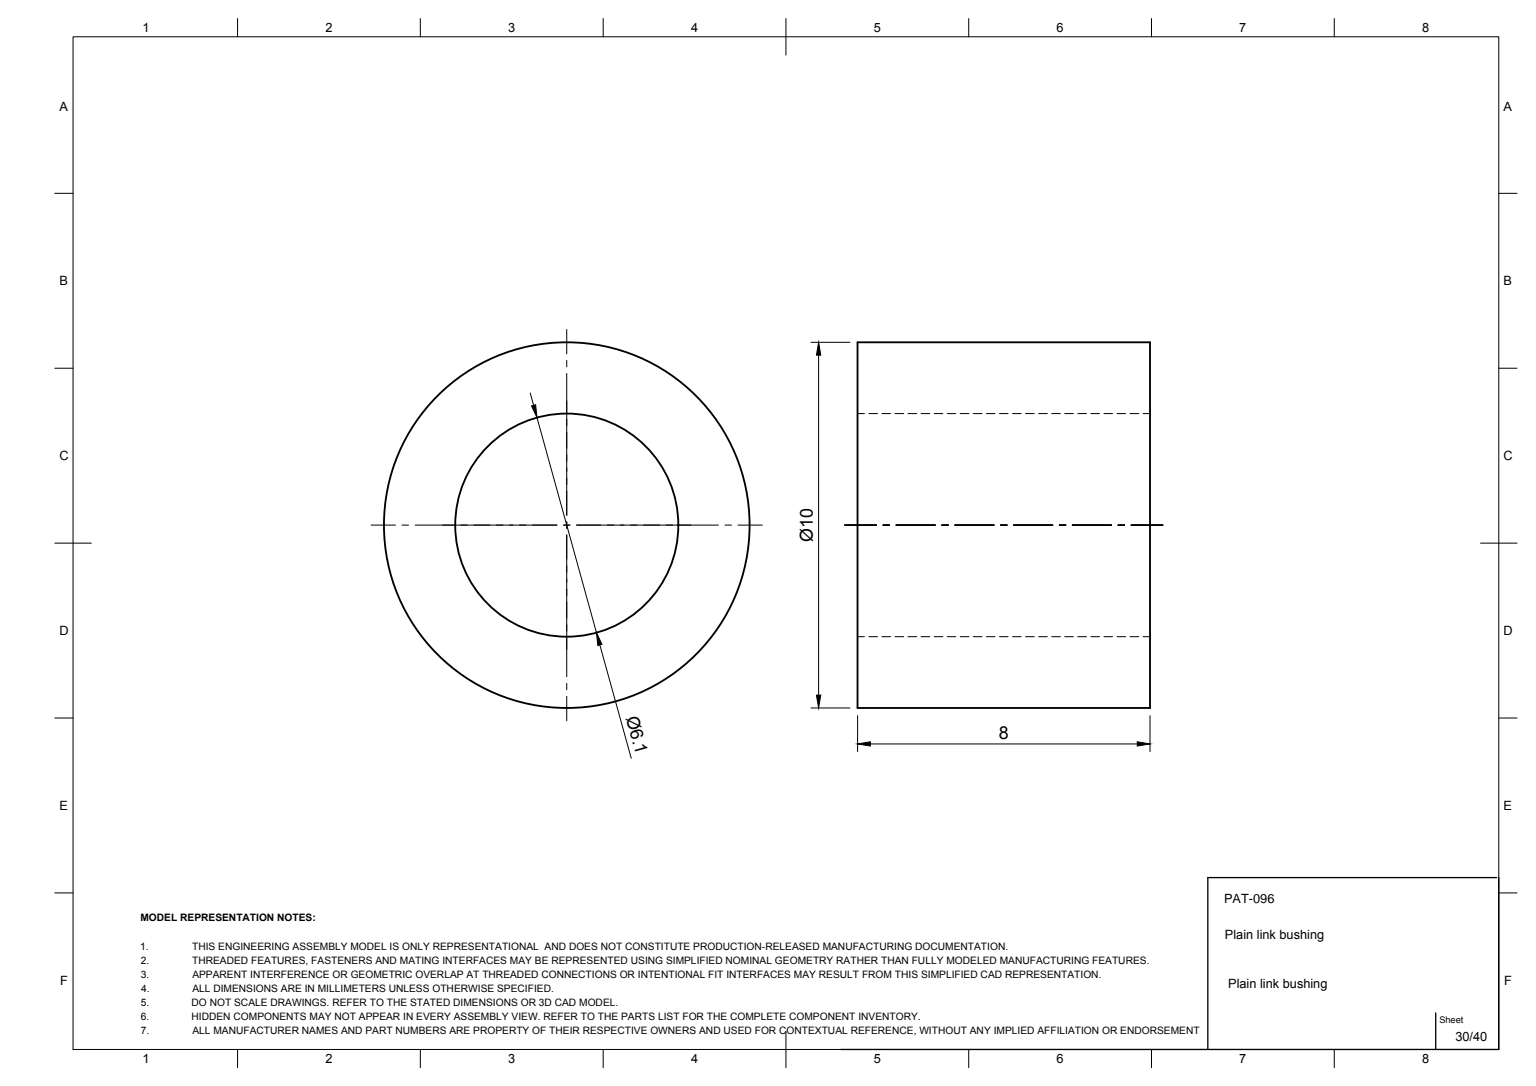
ISO-10303-21;
HEADER;
/* Generated by software containing ST-Developer
 * from STEP Tools, Inc. (www.steptools.com) 
 */

FILE_DESCRIPTION(
/* description */ ('PAT-096'),
/* implementation_level */ '2;1');

FILE_NAME(
/* name */ 'Plain link bushing.step',
/* time_stamp */ '2026-10-29T17:03:14-07:00',
/* author */ (''),
/* organization */ (''),
/* preprocessor_version */ 'ST-DEVELOPER v20.2',
/* originating_system */ 'Autodesk Translation Framework v15.17.0.0',
/* authorisation */ '');

FILE_SCHEMA (('AUTOMOTIVE_DESIGN { 1 0 10303 214 3 1 1 }'));
ENDSEC;

DATA;
#10=MECHANICAL_DESIGN_GEOMETRIC_PRESENTATION_REPRESENTATION('',(#427),#10650);
#357=SHAPE_REPRESENTATION_RELATIONSHIP('SRR','None',#10820,#388);
#388=ADVANCED_BREP_SHAPE_REPRESENTATION('',(#464),#10638);
#427=STYLED_ITEM('',(#11057),#464);
#464=MANIFOLD_SOLID_BREP('Body1',#5562);
#568=FACE_BOUND('',#1470,.T.);
#569=FACE_BOUND('',#1472,.T.);
#736=PLANE('',#6443);
#737=PLANE('',#6444);
#1036=FACE_OUTER_BOUND('',#1467,.T.);
#1037=FACE_OUTER_BOUND('',#1468,.T.);
#1038=FACE_OUTER_BOUND('',#1469,.T.);
#1039=FACE_OUTER_BOUND('',#1471,.T.);
#1467=EDGE_LOOP('',(#4731,#4732,#4733,#4734));
#1468=EDGE_LOOP('',(#4735,#4736,#4737,#4738));
#1469=EDGE_LOOP('',(#4739));
#1470=EDGE_LOOP('',(#4740));
#1471=EDGE_LOOP('',(#4741));
#1472=EDGE_LOOP('',(#4742));
#1834=LINE('',#10134,#2163);
#1835=LINE('',#10140,#2164);
#2163=VECTOR('',#7952,0.305);
#2164=VECTOR('',#7959,0.5);
#2503=CIRCLE('',#6438,0.305);
#2504=CIRCLE('',#6439,0.305);
#2505=CIRCLE('',#6441,0.5);
#2506=CIRCLE('',#6442,0.5);
#2923=VERTEX_POINT('',#10131);
#2924=VERTEX_POINT('',#10133);
#2925=VERTEX_POINT('',#10137);
#2926=VERTEX_POINT('',#10139);
#3544=EDGE_CURVE('',#2923,#2923,#2503,.T.);
#3545=EDGE_CURVE('',#2923,#2924,#1834,.T.);
#3546=EDGE_CURVE('',#2924,#2924,#2504,.T.);
#3547=EDGE_CURVE('',#2925,#2925,#2505,.T.);
#3548=EDGE_CURVE('',#2925,#2926,#1835,.T.);
#3549=EDGE_CURVE('',#2926,#2926,#2506,.T.);
#4731=ORIENTED_EDGE('',*,*,#3544,.F.);
#4732=ORIENTED_EDGE('',*,*,#3545,.T.);
#4733=ORIENTED_EDGE('',*,*,#3546,.T.);
#4734=ORIENTED_EDGE('',*,*,#3545,.F.);
#4735=ORIENTED_EDGE('',*,*,#3547,.F.);
#4736=ORIENTED_EDGE('',*,*,#3548,.T.);
#4737=ORIENTED_EDGE('',*,*,#3549,.T.);
#4738=ORIENTED_EDGE('',*,*,#3548,.F.);
#4739=ORIENTED_EDGE('',*,*,#3547,.T.);
#4740=ORIENTED_EDGE('',*,*,#3544,.T.);
#4741=ORIENTED_EDGE('',*,*,#3549,.F.);
#4742=ORIENTED_EDGE('',*,*,#3546,.F.);
#5162=CYLINDRICAL_SURFACE('',#6437,0.305);
#5163=CYLINDRICAL_SURFACE('',#6440,0.5);
#5441=ADVANCED_FACE('',(#1036),#5162,.F.);
#5442=ADVANCED_FACE('',(#1037),#5163,.T.);
#5443=ADVANCED_FACE('',(#1038,#568),#736,.T.);
#5444=ADVANCED_FACE('',(#1039,#569),#737,.F.);
#5562=CLOSED_SHELL('',(#5441,#5442,#5443,#5444));
#6436=AXIS2_PLACEMENT_3D('',#10129,#7946,#7947);
#6437=AXIS2_PLACEMENT_3D('',#10130,#7948,#7949);
#6438=AXIS2_PLACEMENT_3D('',#10132,#7950,#7951);
#6439=AXIS2_PLACEMENT_3D('',#10135,#7953,#7954);
#6440=AXIS2_PLACEMENT_3D('',#10136,#7955,#7956);
#6441=AXIS2_PLACEMENT_3D('',#10138,#7957,#7958);
#6442=AXIS2_PLACEMENT_3D('',#10141,#7960,#7961);
#6443=AXIS2_PLACEMENT_3D('',#10142,#7962,#7963);
#6444=AXIS2_PLACEMENT_3D('',#10143,#7964,#7965);
#7946=DIRECTION('axis',(0.,0.,1.));
#7947=DIRECTION('refdir',(1.,0.,0.));
#7948=DIRECTION('center_axis',(0.,0.,1.));
#7949=DIRECTION('ref_axis',(1.,0.,0.));
#7950=DIRECTION('center_axis',(0.,0.,-1.));
#7951=DIRECTION('ref_axis',(1.,0.,0.));
#7952=DIRECTION('',(0.,0.,-1.));
#7953=DIRECTION('center_axis',(0.,0.,-1.));
#7954=DIRECTION('ref_axis',(1.,0.,0.));
#7955=DIRECTION('center_axis',(0.,0.,1.));
#7956=DIRECTION('ref_axis',(1.,0.,0.));
#7957=DIRECTION('center_axis',(0.,0.,1.));
#7958=DIRECTION('ref_axis',(1.,0.,0.));
#7959=DIRECTION('',(0.,0.,-1.));
#7960=DIRECTION('center_axis',(0.,0.,1.));
#7961=DIRECTION('ref_axis',(1.,0.,0.));
#7962=DIRECTION('center_axis',(0.,0.,1.));
#7963=DIRECTION('ref_axis',(1.,0.,0.));
#7964=DIRECTION('center_axis',(0.,0.,1.));
#7965=DIRECTION('ref_axis',(1.,0.,0.));
#10129=CARTESIAN_POINT('',(0.,0.,0.));
#10130=CARTESIAN_POINT('Origin',(0.,2.,8.8));
#10131=CARTESIAN_POINT('',(-0.305,2.,9.6));
#10132=CARTESIAN_POINT('Origin',(0.,2.,9.6));
#10133=CARTESIAN_POINT('',(-0.305,2.,8.8));
#10134=CARTESIAN_POINT('',(-0.305,2.,8.8));
#10135=CARTESIAN_POINT('Origin',(0.,2.,8.8));
#10136=CARTESIAN_POINT('Origin',(0.,2.,8.8));
#10137=CARTESIAN_POINT('',(-0.5,2.,9.6));
#10138=CARTESIAN_POINT('Origin',(0.,2.,9.6));
#10139=CARTESIAN_POINT('',(-0.5,2.,8.8));
#10140=CARTESIAN_POINT('',(-0.5,2.,8.8));
#10141=CARTESIAN_POINT('Origin',(0.,2.,8.8));
#10142=CARTESIAN_POINT('Origin',(0.,2.,9.6));
#10143=CARTESIAN_POINT('Origin',(0.,2.,8.8));
#10599=UNCERTAINTY_MEASURE_WITH_UNIT(LENGTH_MEASURE(0.001),#10651,
'DISTANCE_ACCURACY_VALUE',
'Maximum model space distance between geometric entities at asserted c
onnectivities');
#10611=UNCERTAINTY_MEASURE_WITH_UNIT(LENGTH_MEASURE(0.001),#10651,
'DISTANCE_ACCURACY_VALUE',
'Maximum model space distance between geometric entities at asserted c
onnectivities');
#10638=(
GEOMETRIC_REPRESENTATION_CONTEXT(3)
GLOBAL_UNCERTAINTY_ASSIGNED_CONTEXT((#10599))
GLOBAL_UNIT_ASSIGNED_CONTEXT((#10651,#10653,#10654))
REPRESENTATION_CONTEXT('','3D')
);
#10650=(
GEOMETRIC_REPRESENTATION_CONTEXT(3)
GLOBAL_UNCERTAINTY_ASSIGNED_CONTEXT((#10611))
GLOBAL_UNIT_ASSIGNED_CONTEXT((#10651,#10653,#10654))
REPRESENTATION_CONTEXT('','3D')
);
#10651=(
LENGTH_UNIT()
NAMED_UNIT(*)
SI_UNIT(.CENTI.,.METRE.)
);
#10653=(
NAMED_UNIT(*)
PLANE_ANGLE_UNIT()
SI_UNIT($,.RADIAN.)
);
#10654=(
NAMED_UNIT(*)
SI_UNIT($,.STERADIAN.)
SOLID_ANGLE_UNIT()
);
#10681=SHAPE_DEFINITION_REPRESENTATION(#10724,#10820);
#10724=PRODUCT_DEFINITION_SHAPE('',$,#10859);
#10820=SHAPE_REPRESENTATION('',(#6436),#10638);
#10832=PRODUCT_DEFINITION_CONTEXT('part definition',#10948,'design');
#10859=PRODUCT_DEFINITION('Plain link bushing','Plain link bushing',#10897,
#10832);
#10897=PRODUCT_DEFINITION_FORMATION('',$,#10976);
#10948=APPLICATION_CONTEXT(
'Core Data for Automotive Mechanical Design Process');
#10949=PRODUCT_CONTEXT('part definition',#10948,'mechanical');
#10976=PRODUCT('Plain link bushing','Plain link bushing',
'Plain link bushing',(#10949));
#11051=COLOUR_RGB('Sky Blue',0.24,0.69,0.87);
#11052=FILL_AREA_STYLE_COLOUR('',#11051);
#11053=FILL_AREA_STYLE('',(#11052));
#11054=SURFACE_STYLE_FILL_AREA(#11053);
#11055=SURFACE_SIDE_STYLE('',(#11054));
#11056=SURFACE_STYLE_USAGE(.BOTH.,#11055);
#11057=PRESENTATION_STYLE_ASSIGNMENT((#11056));
ENDSEC;
END-ISO-10303-21;
